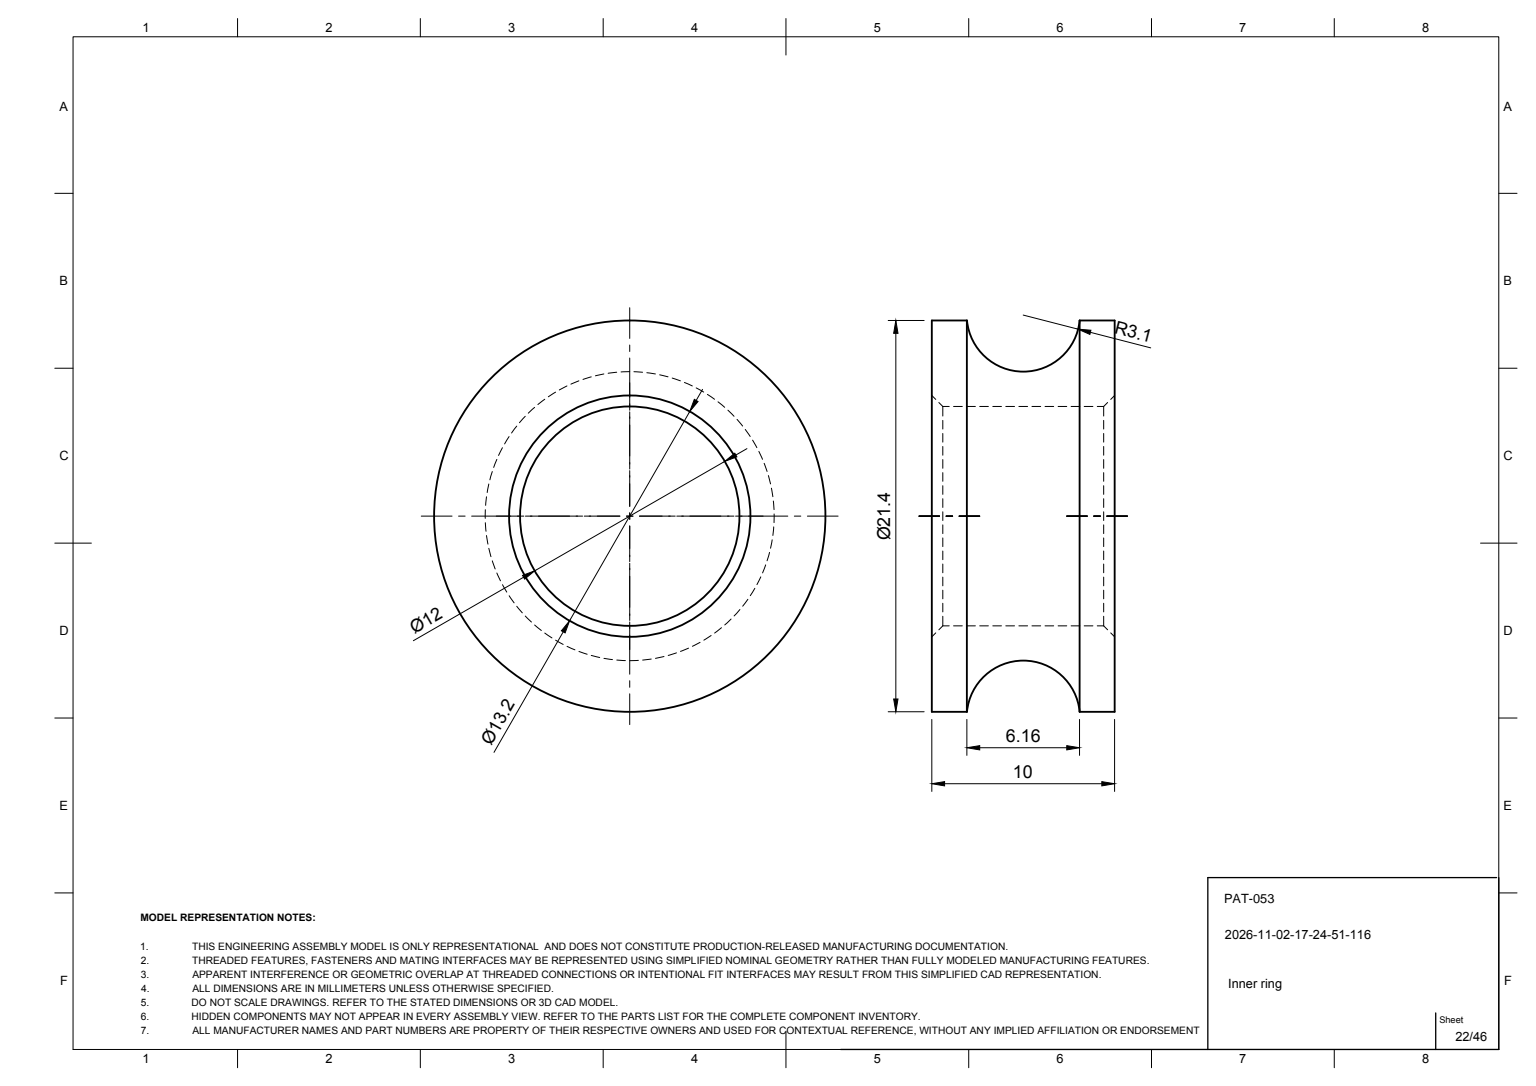
ISO-10303-21;
HEADER;
/* Generated by software containing ST-Developer
 * from STEP Tools, Inc. (www.steptools.com) 
 */

FILE_DESCRIPTION(
/* description */ ('Hand-operated arbor press'),
/* implementation_level */ '2;1');

FILE_NAME(
/* name */ 'Inner ring.step',
/* time_stamp */ '2026-10-28T03:25:25-07:00',
/* author */ (''),
/* organization */ (''),
/* preprocessor_version */ 'ST-DEVELOPER v20.2',
/* originating_system */ 'Autodesk Translation Framework v15.17.0.0',
/* authorisation */ '');

FILE_SCHEMA (('AUTOMOTIVE_DESIGN { 1 0 10303 214 3 1 1 }'));
ENDSEC;

DATA;
#10=MECHANICAL_DESIGN_GEOMETRIC_PRESENTATION_REPRESENTATION('',(#602),#32751);
#471=TOROIDAL_SURFACE('',#13416,1.1,0.309556);
#481=CONICAL_SURFACE('',#13427,0.63,0.785398163397448);
#482=CONICAL_SURFACE('',#13434,0.63,0.785398163397448);
#518=SHAPE_REPRESENTATION_RELATIONSHIP('SRR','None',#32948,#560);
#560=ADVANCED_BREP_SHAPE_REPRESENTATION('',(#650),#32722);
#602=STYLED_ITEM('',(#33242),#650);
#650=MANIFOLD_SOLID_BREP('Body1',#12500);
#802=FACE_BOUND('',#2320,.T.);
#803=FACE_BOUND('',#2323,.T.);
#977=PLANE('',#13429);
#978=PLANE('',#13432);
#1512=FACE_OUTER_BOUND('',#2315,.T.);
#1513=FACE_OUTER_BOUND('',#2316,.T.);
#1514=FACE_OUTER_BOUND('',#2317,.T.);
#1515=FACE_OUTER_BOUND('',#2318,.T.);
#1516=FACE_OUTER_BOUND('',#2319,.T.);
#1517=FACE_OUTER_BOUND('',#2321,.T.);
#1518=FACE_OUTER_BOUND('',#2322,.T.);
#1519=FACE_OUTER_BOUND('',#2324,.T.);
#2315=EDGE_LOOP('',(#9342,#9343,#9344,#9345,#9346,#9347));
#2316=EDGE_LOOP('',(#9348,#9349,#9350,#9351,#9352));
#2317=EDGE_LOOP('',(#9353,#9354,#9355,#9356));
#2318=EDGE_LOOP('',(#9357,#9358,#9359,#9360));
#2319=EDGE_LOOP('',(#9361));
#2320=EDGE_LOOP('',(#9362));
#2321=EDGE_LOOP('',(#9363,#9364,#9365,#9366,#9367));
#2322=EDGE_LOOP('',(#9368));
#2323=EDGE_LOOP('',(#9369));
#2324=EDGE_LOOP('',(#9370,#9371,#9372,#9373));
#3155=LINE('',#18736,#4326);
#3156=LINE('',#18742,#4327);
#3157=LINE('',#18746,#4328);
#3158=LINE('',#18752,#4329);
#3159=LINE('',#18757,#4330);
#4326=VECTOR('',#15334,1.070235);
#4327=VECTOR('',#15341,0.6);
#4328=VECTOR('',#15346,0.63);
#4329=VECTOR('',#15355,1.070235);
#4330=VECTOR('',#15362,0.63);
#5344=CIRCLE('',#13417,1.070235);
#5345=CIRCLE('',#13418,1.070235);
#5346=CIRCLE('',#13419,0.309556);
#5347=CIRCLE('',#13420,1.070235);
#5348=CIRCLE('',#13421,1.070235);
#5349=CIRCLE('',#13423,1.070235);
#5350=CIRCLE('',#13425,0.6);
#5351=CIRCLE('',#13426,0.6);
#5352=CIRCLE('',#13428,0.66);
#5353=CIRCLE('',#13431,1.070235);
#5354=CIRCLE('',#13433,0.66);
#5894=VERTEX_POINT('',#18725);
#5895=VERTEX_POINT('',#18726);
#5896=VERTEX_POINT('',#18729);
#5897=VERTEX_POINT('',#18731);
#5898=VERTEX_POINT('',#18735);
#5899=VERTEX_POINT('',#18739);
#5900=VERTEX_POINT('',#18741);
#5901=VERTEX_POINT('',#18745);
#5902=VERTEX_POINT('',#18750);
#5903=VERTEX_POINT('',#18754);
#7174=EDGE_CURVE('',#5894,#5895,#5344,.T.);
#7175=EDGE_CURVE('',#5895,#5894,#5345,.T.);
#7176=EDGE_CURVE('',#5895,#5896,#5346,.T.);
#7177=EDGE_CURVE('',#5897,#5896,#5347,.T.);
#7178=EDGE_CURVE('',#5896,#5897,#5348,.T.);
#7179=EDGE_CURVE('',#5897,#5898,#3155,.T.);
#7180=EDGE_CURVE('',#5898,#5898,#5349,.T.);
#7181=EDGE_CURVE('',#5899,#5899,#5350,.T.);
#7182=EDGE_CURVE('',#5899,#5900,#3156,.T.);
#7183=EDGE_CURVE('',#5900,#5900,#5351,.T.);
#7184=EDGE_CURVE('',#5900,#5901,#3157,.T.);
#7185=EDGE_CURVE('',#5901,#5901,#5352,.T.);
#7186=EDGE_CURVE('',#5902,#5902,#5353,.T.);
#7187=EDGE_CURVE('',#5902,#5894,#3158,.T.);
#7188=EDGE_CURVE('',#5903,#5903,#5354,.T.);
#7189=EDGE_CURVE('',#5903,#5899,#3159,.T.);
#9342=ORIENTED_EDGE('',*,*,#7174,.F.);
#9343=ORIENTED_EDGE('',*,*,#7175,.F.);
#9344=ORIENTED_EDGE('',*,*,#7176,.T.);
#9345=ORIENTED_EDGE('',*,*,#7177,.F.);
#9346=ORIENTED_EDGE('',*,*,#7178,.F.);
#9347=ORIENTED_EDGE('',*,*,#7176,.F.);
#9348=ORIENTED_EDGE('',*,*,#7177,.T.);
#9349=ORIENTED_EDGE('',*,*,#7178,.T.);
#9350=ORIENTED_EDGE('',*,*,#7179,.T.);
#9351=ORIENTED_EDGE('',*,*,#7180,.T.);
#9352=ORIENTED_EDGE('',*,*,#7179,.F.);
#9353=ORIENTED_EDGE('',*,*,#7181,.T.);
#9354=ORIENTED_EDGE('',*,*,#7182,.T.);
#9355=ORIENTED_EDGE('',*,*,#7183,.F.);
#9356=ORIENTED_EDGE('',*,*,#7182,.F.);
#9357=ORIENTED_EDGE('',*,*,#7183,.T.);
#9358=ORIENTED_EDGE('',*,*,#7184,.T.);
#9359=ORIENTED_EDGE('',*,*,#7185,.F.);
#9360=ORIENTED_EDGE('',*,*,#7184,.F.);
#9361=ORIENTED_EDGE('',*,*,#7180,.F.);
#9362=ORIENTED_EDGE('',*,*,#7185,.T.);
#9363=ORIENTED_EDGE('',*,*,#7186,.F.);
#9364=ORIENTED_EDGE('',*,*,#7187,.T.);
#9365=ORIENTED_EDGE('',*,*,#7174,.T.);
#9366=ORIENTED_EDGE('',*,*,#7175,.T.);
#9367=ORIENTED_EDGE('',*,*,#7187,.F.);
#9368=ORIENTED_EDGE('',*,*,#7186,.T.);
#9369=ORIENTED_EDGE('',*,*,#7188,.F.);
#9370=ORIENTED_EDGE('',*,*,#7188,.T.);
#9371=ORIENTED_EDGE('',*,*,#7189,.T.);
#9372=ORIENTED_EDGE('',*,*,#7181,.F.);
#9373=ORIENTED_EDGE('',*,*,#7189,.F.);
#11729=CYLINDRICAL_SURFACE('',#13422,1.070235);
#11730=CYLINDRICAL_SURFACE('',#13424,0.6);
#11731=CYLINDRICAL_SURFACE('',#13430,1.070235);
#12021=ADVANCED_FACE('',(#1512),#471,.F.);
#12022=ADVANCED_FACE('',(#1513),#11729,.T.);
#12023=ADVANCED_FACE('',(#1514),#11730,.F.);
#12024=ADVANCED_FACE('',(#1515),#481,.F.);
#12025=ADVANCED_FACE('',(#1516,#802),#977,.T.);
#12026=ADVANCED_FACE('',(#1517),#11731,.T.);
#12027=ADVANCED_FACE('',(#1518,#803),#978,.T.);
#12028=ADVANCED_FACE('',(#1519),#482,.F.);
#12500=CLOSED_SHELL('',(#12021,#12022,#12023,#12024,#12025,#12026,#12027,
#12028));
#13415=AXIS2_PLACEMENT_3D('',#18723,#15318,#15319);
#13416=AXIS2_PLACEMENT_3D('',#18724,#15320,#15321);
#13417=AXIS2_PLACEMENT_3D('',#18727,#15322,#15323);
#13418=AXIS2_PLACEMENT_3D('',#18728,#15324,#15325);
#13419=AXIS2_PLACEMENT_3D('',#18730,#15326,#15327);
#13420=AXIS2_PLACEMENT_3D('',#18732,#15328,#15329);
#13421=AXIS2_PLACEMENT_3D('',#18733,#15330,#15331);
#13422=AXIS2_PLACEMENT_3D('',#18734,#15332,#15333);
#13423=AXIS2_PLACEMENT_3D('',#18737,#15335,#15336);
#13424=AXIS2_PLACEMENT_3D('',#18738,#15337,#15338);
#13425=AXIS2_PLACEMENT_3D('',#18740,#15339,#15340);
#13426=AXIS2_PLACEMENT_3D('',#18743,#15342,#15343);
#13427=AXIS2_PLACEMENT_3D('',#18744,#15344,#15345);
#13428=AXIS2_PLACEMENT_3D('',#18747,#15347,#15348);
#13429=AXIS2_PLACEMENT_3D('',#18748,#15349,#15350);
#13430=AXIS2_PLACEMENT_3D('',#18749,#15351,#15352);
#13431=AXIS2_PLACEMENT_3D('',#18751,#15353,#15354);
#13432=AXIS2_PLACEMENT_3D('',#18753,#15356,#15357);
#13433=AXIS2_PLACEMENT_3D('',#18755,#15358,#15359);
#13434=AXIS2_PLACEMENT_3D('',#18756,#15360,#15361);
#15318=DIRECTION('axis',(0.,0.,1.));
#15319=DIRECTION('refdir',(1.,0.,0.));
#15320=DIRECTION('center_axis',(0.,-1.,0.));
#15321=DIRECTION('ref_axis',(0.,0.,-1.));
#15322=DIRECTION('center_axis',(0.,-1.,0.));
#15323=DIRECTION('ref_axis',(1.,0.,0.));
#15324=DIRECTION('center_axis',(0.,-1.,0.));
#15325=DIRECTION('ref_axis',(1.,0.,0.));
#15326=DIRECTION('center_axis',(1.,0.,1.22464679914735E-16));
#15327=DIRECTION('ref_axis',(-1.22464679914735E-16,0.,1.));
#15328=DIRECTION('center_axis',(0.,1.,0.));
#15329=DIRECTION('ref_axis',(1.,0.,0.));
#15330=DIRECTION('center_axis',(0.,1.,0.));
#15331=DIRECTION('ref_axis',(1.,0.,0.));
#15332=DIRECTION('center_axis',(0.,-1.,0.));
#15333=DIRECTION('ref_axis',(1.,0.,0.));
#15334=DIRECTION('',(0.,1.,0.));
#15335=DIRECTION('center_axis',(0.,-1.,0.));
#15336=DIRECTION('ref_axis',(1.,0.,0.));
#15337=DIRECTION('center_axis',(0.,-1.,0.));
#15338=DIRECTION('ref_axis',(1.,0.,0.));
#15339=DIRECTION('center_axis',(0.,-1.,0.));
#15340=DIRECTION('ref_axis',(1.,0.,0.));
#15341=DIRECTION('',(0.,1.,0.));
#15342=DIRECTION('center_axis',(0.,-1.,0.));
#15343=DIRECTION('ref_axis',(1.,0.,0.));
#15344=DIRECTION('center_axis',(0.,1.,0.));
#15345=DIRECTION('ref_axis',(1.,0.,0.));
#15346=DIRECTION('',(-0.707106781186548,0.707106781186547,-8.65956056235493E-17));
#15347=DIRECTION('center_axis',(0.,-1.,0.));
#15348=DIRECTION('ref_axis',(1.,0.,0.));
#15349=DIRECTION('center_axis',(0.,1.,0.));
#15350=DIRECTION('ref_axis',(0.,0.,1.));
#15351=DIRECTION('center_axis',(0.,-1.,0.));
#15352=DIRECTION('ref_axis',(1.,0.,0.));
#15353=DIRECTION('center_axis',(0.,-1.,0.));
#15354=DIRECTION('ref_axis',(1.,0.,0.));
#15355=DIRECTION('',(0.,1.,0.));
#15356=DIRECTION('center_axis',(0.,-1.,0.));
#15357=DIRECTION('ref_axis',(0.,0.,-1.));
#15358=DIRECTION('center_axis',(0.,-1.,0.));
#15359=DIRECTION('ref_axis',(1.,0.,0.));
#15360=DIRECTION('center_axis',(0.,-1.,0.));
#15361=DIRECTION('ref_axis',(1.,0.,0.));
#15362=DIRECTION('',(0.707106781186548,0.707106781186547,8.65956056235493E-17));
#18723=CARTESIAN_POINT('',(0.,0.,0.));
#18724=CARTESIAN_POINT('Origin',(0.,0.,0.));
#18725=CARTESIAN_POINT('',(-1.070235,-0.308121667383195,-1.31065986708547E-16));
#18726=CARTESIAN_POINT('',(-1.31065986708547E-16,-0.308121667383195,1.070235));
#18727=CARTESIAN_POINT('Origin',(0.,-0.308121667383195,0.));
#18728=CARTESIAN_POINT('Origin',(0.,-0.308121667383195,0.));
#18729=CARTESIAN_POINT('',(-1.31065986708547E-16,0.308121667383195,1.070235));
#18730=CARTESIAN_POINT('Origin',(-1.34711147906209E-16,0.,1.1));
#18731=CARTESIAN_POINT('',(-1.070235,0.308121667383195,1.31065986708547E-16));
#18732=CARTESIAN_POINT('Origin',(0.,0.308121667383195,0.));
#18733=CARTESIAN_POINT('Origin',(0.,0.308121667383195,0.));
#18734=CARTESIAN_POINT('Origin',(0.,0.,0.));
#18735=CARTESIAN_POINT('',(-1.070235,0.5,-1.31065986708547E-16));
#18736=CARTESIAN_POINT('',(-1.070235,0.,-1.31065986708547E-16));
#18737=CARTESIAN_POINT('Origin',(0.,0.5,0.));
#18738=CARTESIAN_POINT('Origin',(0.,0.,0.));
#18739=CARTESIAN_POINT('',(-0.6,-0.44,-7.34788079488412E-17));
#18740=CARTESIAN_POINT('Origin',(0.,-0.44,0.));
#18741=CARTESIAN_POINT('',(-0.6,0.44,-7.34788079488412E-17));
#18742=CARTESIAN_POINT('',(-0.6,0.,-7.34788079488412E-17));
#18743=CARTESIAN_POINT('Origin',(0.,0.44,0.));
#18744=CARTESIAN_POINT('Origin',(0.,0.47,0.));
#18745=CARTESIAN_POINT('',(-0.66,0.5,-8.08266887437253E-17));
#18746=CARTESIAN_POINT('',(-0.63,0.47,-7.71527483462832E-17));
#18747=CARTESIAN_POINT('Origin',(0.,0.5,0.));
#18748=CARTESIAN_POINT('Origin',(1.070235,0.5,0.));
#18749=CARTESIAN_POINT('Origin',(0.,0.,0.));
#18750=CARTESIAN_POINT('',(-1.070235,-0.5,-1.31065986708547E-16));
#18751=CARTESIAN_POINT('Origin',(0.,-0.5,0.));
#18752=CARTESIAN_POINT('',(-1.070235,0.,-1.31065986708547E-16));
#18753=CARTESIAN_POINT('Origin',(0.66,-0.5,0.));
#18754=CARTESIAN_POINT('',(-0.66,-0.5,-8.08266887437253E-17));
#18755=CARTESIAN_POINT('Origin',(0.,-0.5,0.));
#18756=CARTESIAN_POINT('Origin',(0.,-0.47,0.));
#18757=CARTESIAN_POINT('',(-0.63,-0.47,-7.71527483462832E-17));
#32673=UNCERTAINTY_MEASURE_WITH_UNIT(LENGTH_MEASURE(0.001),#32752,
'DISTANCE_ACCURACY_VALUE',
'Maximum model space distance between geometric entities at asserted c
onnectivities');
#32702=UNCERTAINTY_MEASURE_WITH_UNIT(LENGTH_MEASURE(0.001),#32752,
'DISTANCE_ACCURACY_VALUE',
'Maximum model space distance between geometric entities at asserted c
onnectivities');
#32722=(
GEOMETRIC_REPRESENTATION_CONTEXT(3)
GLOBAL_UNCERTAINTY_ASSIGNED_CONTEXT((#32673))
GLOBAL_UNIT_ASSIGNED_CONTEXT((#32752,#32754,#32755))
REPRESENTATION_CONTEXT('','3D')
);
#32751=(
GEOMETRIC_REPRESENTATION_CONTEXT(3)
GLOBAL_UNCERTAINTY_ASSIGNED_CONTEXT((#32702))
GLOBAL_UNIT_ASSIGNED_CONTEXT((#32752,#32754,#32755))
REPRESENTATION_CONTEXT('','3D')
);
#32752=(
LENGTH_UNIT()
NAMED_UNIT(*)
SI_UNIT(.CENTI.,.METRE.)
);
#32754=(
NAMED_UNIT(*)
PLANE_ANGLE_UNIT()
SI_UNIT($,.RADIAN.)
);
#32755=(
NAMED_UNIT(*)
SI_UNIT($,.STERADIAN.)
SOLID_ANGLE_UNIT()
);
#32775=SHAPE_DEFINITION_REPRESENTATION(#32823,#32948);
#32823=PRODUCT_DEFINITION_SHAPE('',$,#32997);
#32948=SHAPE_REPRESENTATION('',(#13415),#32722);
#32977=PRODUCT_DEFINITION_CONTEXT('part definition',#33123,'design');
#32997=PRODUCT_DEFINITION('Inner ring','Inner ring',#33045,#32977);
#33045=PRODUCT_DEFINITION_FORMATION('',$,#33144);
#33123=APPLICATION_CONTEXT(
'Core Data for Automotive Mechanical Design Process');
#33124=PRODUCT_CONTEXT('part definition',#33123,'mechanical');
#33144=PRODUCT('Inner ring','Inner ring','Inner ring',(#33124));
#33236=COLOUR_RGB('Grey',0.48,0.52,0.57);
#33237=FILL_AREA_STYLE_COLOUR('',#33236);
#33238=FILL_AREA_STYLE('',(#33237));
#33239=SURFACE_STYLE_FILL_AREA(#33238);
#33240=SURFACE_SIDE_STYLE('',(#33239));
#33241=SURFACE_STYLE_USAGE(.BOTH.,#33240);
#33242=PRESENTATION_STYLE_ASSIGNMENT((#33241));
ENDSEC;
END-ISO-10303-21;
